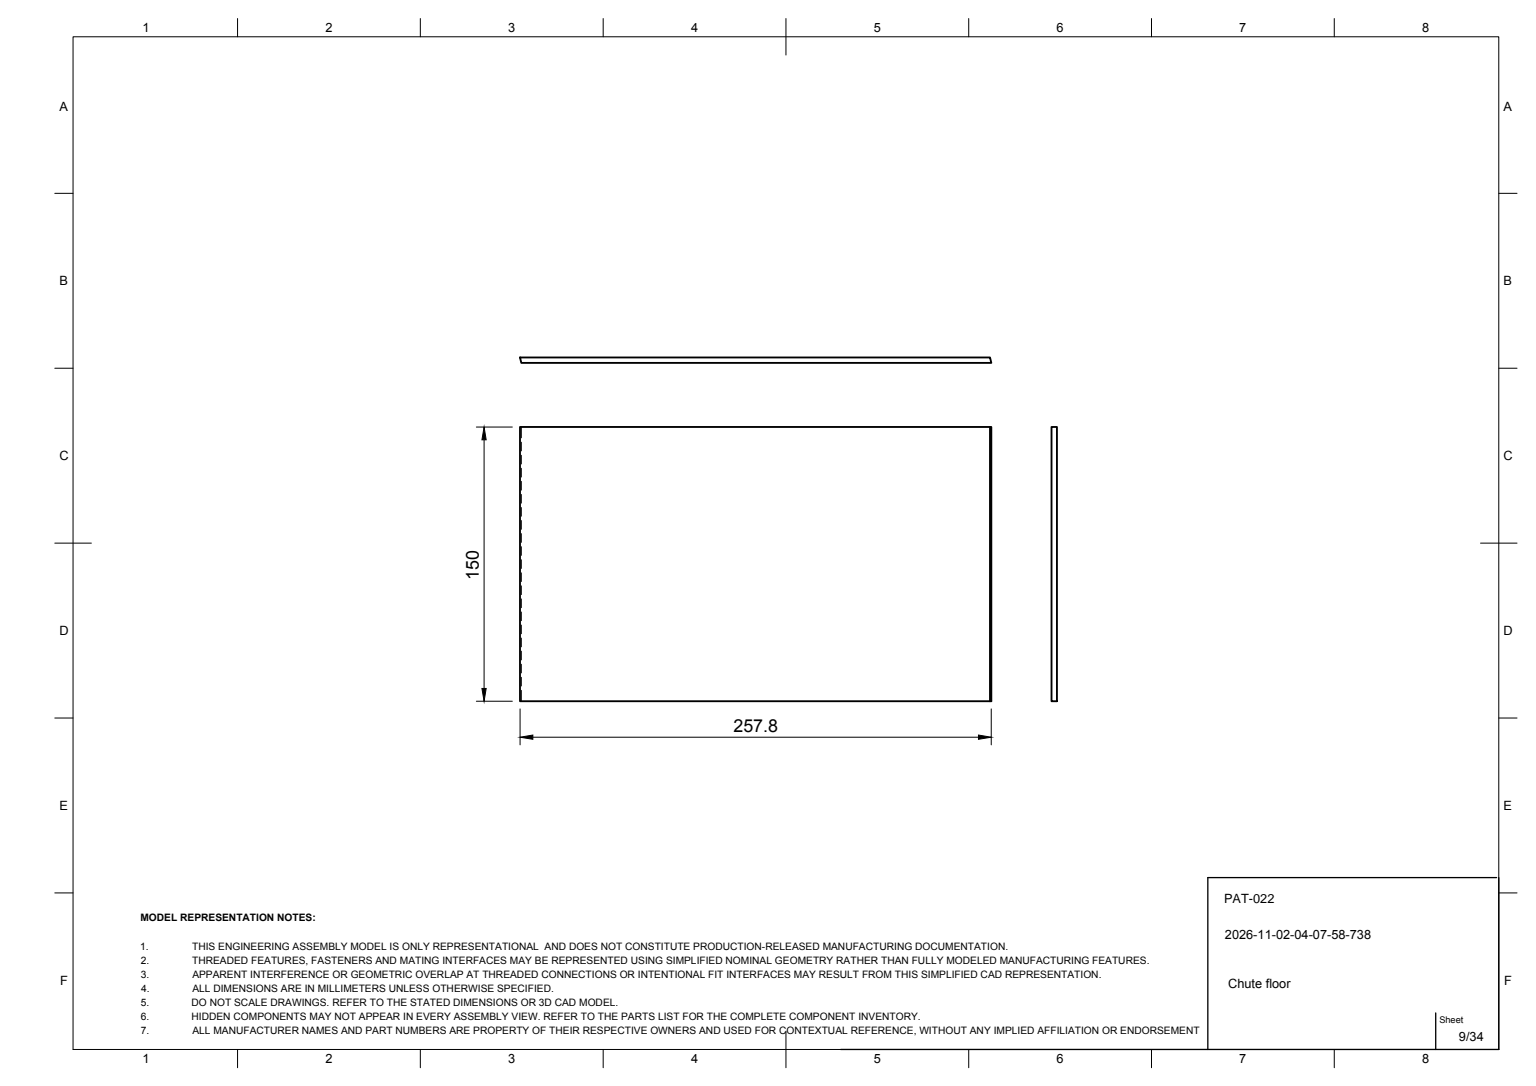
ISO-10303-21;
HEADER;
/* Generated by software containing ST-Developer
 * from STEP Tools, Inc. (www.steptools.com) 
 */

FILE_DESCRIPTION(
/* description */ ('Chute with adjustable gate'),
/* implementation_level */ '2;1');

FILE_NAME(
/* name */ 'Chute floor.step',
/* time_stamp */ '2026-10-27T10:52:28-07:00',
/* author */ (''),
/* organization */ (''),
/* preprocessor_version */ 'ST-DEVELOPER v20.2',
/* originating_system */ 'Autodesk Translation Framework v15.17.0.0',
/* authorisation */ '');

FILE_SCHEMA (('AUTOMOTIVE_DESIGN { 1 0 10303 214 3 1 1 }'));
ENDSEC;

DATA;
#10=MECHANICAL_DESIGN_GEOMETRIC_PRESENTATION_REPRESENTATION('',(#418),#13094);
#354=SHAPE_REPRESENTATION_RELATIONSHIP('SRR','None',#13255,#386);
#386=ADVANCED_BREP_SHAPE_REPRESENTATION('',(#450),#13064);
#418=STYLED_ITEM('',(#13481),#450);
#450=MANIFOLD_SOLID_BREP('Body1',#7601);
#618=PLANE('',#8045);
#619=PLANE('',#8046);
#620=PLANE('',#8047);
#621=PLANE('',#8048);
#622=PLANE('',#8049);
#623=PLANE('',#8050);
#950=FACE_OUTER_BOUND('',#1383,.T.);
#951=FACE_OUTER_BOUND('',#1384,.T.);
#952=FACE_OUTER_BOUND('',#1385,.T.);
#953=FACE_OUTER_BOUND('',#1386,.T.);
#954=FACE_OUTER_BOUND('',#1387,.T.);
#955=FACE_OUTER_BOUND('',#1388,.T.);
#1383=EDGE_LOOP('',(#5354,#5355,#5356,#5357));
#1384=EDGE_LOOP('',(#5358,#5359,#5360,#5361));
#1385=EDGE_LOOP('',(#5362,#5363,#5364,#5365));
#1386=EDGE_LOOP('',(#5366,#5367,#5368,#5369));
#1387=EDGE_LOOP('',(#5370,#5371,#5372,#5373));
#1388=EDGE_LOOP('',(#5374,#5375,#5376,#5377));
#1928=LINE('',#11085,#2705);
#1929=LINE('',#11087,#2706);
#1930=LINE('',#11089,#2707);
#1931=LINE('',#11090,#2708);
#1932=LINE('',#11093,#2709);
#1933=LINE('',#11095,#2710);
#1934=LINE('',#11096,#2711);
#1935=LINE('',#11099,#2712);
#1936=LINE('',#11101,#2713);
#1937=LINE('',#11102,#2714);
#1938=LINE('',#11104,#2715);
#1939=LINE('',#11105,#2716);
#2705=VECTOR('',#8886,1.);
#2706=VECTOR('',#8887,1.);
#2707=VECTOR('',#8888,1.);
#2708=VECTOR('',#8889,1.);
#2709=VECTOR('',#8892,1.);
#2710=VECTOR('',#8893,1.);
#2711=VECTOR('',#8894,1.);
#2712=VECTOR('',#8897,1.);
#2713=VECTOR('',#8898,1.);
#2714=VECTOR('',#8899,1.);
#2715=VECTOR('',#8902,1.);
#2716=VECTOR('',#8903,1.);
#3649=VERTEX_POINT('',#11083);
#3650=VERTEX_POINT('',#11084);
#3651=VERTEX_POINT('',#11086);
#3652=VERTEX_POINT('',#11088);
#3653=VERTEX_POINT('',#11092);
#3654=VERTEX_POINT('',#11094);
#3655=VERTEX_POINT('',#11098);
#3656=VERTEX_POINT('',#11100);
#4310=EDGE_CURVE('',#3649,#3650,#1928,.T.);
#4311=EDGE_CURVE('',#3649,#3651,#1929,.T.);
#4312=EDGE_CURVE('',#3652,#3651,#1930,.T.);
#4313=EDGE_CURVE('',#3650,#3652,#1931,.T.);
#4314=EDGE_CURVE('',#3650,#3653,#1932,.T.);
#4315=EDGE_CURVE('',#3654,#3652,#1933,.T.);
#4316=EDGE_CURVE('',#3653,#3654,#1934,.T.);
#4317=EDGE_CURVE('',#3653,#3655,#1935,.T.);
#4318=EDGE_CURVE('',#3656,#3654,#1936,.T.);
#4319=EDGE_CURVE('',#3655,#3656,#1937,.T.);
#4320=EDGE_CURVE('',#3655,#3649,#1938,.T.);
#4321=EDGE_CURVE('',#3651,#3656,#1939,.T.);
#5354=ORIENTED_EDGE('',*,*,#4310,.F.);
#5355=ORIENTED_EDGE('',*,*,#4311,.T.);
#5356=ORIENTED_EDGE('',*,*,#4312,.F.);
#5357=ORIENTED_EDGE('',*,*,#4313,.F.);
#5358=ORIENTED_EDGE('',*,*,#4314,.F.);
#5359=ORIENTED_EDGE('',*,*,#4313,.T.);
#5360=ORIENTED_EDGE('',*,*,#4315,.F.);
#5361=ORIENTED_EDGE('',*,*,#4316,.F.);
#5362=ORIENTED_EDGE('',*,*,#4317,.F.);
#5363=ORIENTED_EDGE('',*,*,#4316,.T.);
#5364=ORIENTED_EDGE('',*,*,#4318,.F.);
#5365=ORIENTED_EDGE('',*,*,#4319,.F.);
#5366=ORIENTED_EDGE('',*,*,#4320,.F.);
#5367=ORIENTED_EDGE('',*,*,#4319,.T.);
#5368=ORIENTED_EDGE('',*,*,#4321,.F.);
#5369=ORIENTED_EDGE('',*,*,#4311,.F.);
#5370=ORIENTED_EDGE('',*,*,#4321,.T.);
#5371=ORIENTED_EDGE('',*,*,#4318,.T.);
#5372=ORIENTED_EDGE('',*,*,#4315,.T.);
#5373=ORIENTED_EDGE('',*,*,#4312,.T.);
#5374=ORIENTED_EDGE('',*,*,#4320,.T.);
#5375=ORIENTED_EDGE('',*,*,#4310,.T.);
#5376=ORIENTED_EDGE('',*,*,#4314,.T.);
#5377=ORIENTED_EDGE('',*,*,#4317,.T.);
#7218=ADVANCED_FACE('',(#950),#618,.T.);
#7219=ADVANCED_FACE('',(#951),#619,.T.);
#7220=ADVANCED_FACE('',(#952),#620,.T.);
#7221=ADVANCED_FACE('',(#953),#621,.T.);
#7222=ADVANCED_FACE('',(#954),#622,.T.);
#7223=ADVANCED_FACE('',(#955),#623,.F.);
#7601=CLOSED_SHELL('',(#7218,#7219,#7220,#7221,#7222,#7223));
#8044=AXIS2_PLACEMENT_3D('',#11081,#8882,#8883);
#8045=AXIS2_PLACEMENT_3D('',#11082,#8884,#8885);
#8046=AXIS2_PLACEMENT_3D('',#11091,#8890,#8891);
#8047=AXIS2_PLACEMENT_3D('',#11097,#8895,#8896);
#8048=AXIS2_PLACEMENT_3D('',#11103,#8900,#8901);
#8049=AXIS2_PLACEMENT_3D('',#11106,#8904,#8905);
#8050=AXIS2_PLACEMENT_3D('',#11107,#8906,#8907);
#8882=DIRECTION('axis',(0.,0.,1.));
#8883=DIRECTION('refdir',(1.,0.,0.));
#8884=DIRECTION('center_axis',(-1.,0.,0.));
#8885=DIRECTION('ref_axis',(0.,0.,1.));
#8886=DIRECTION('',(0.,0.,-1.));
#8887=DIRECTION('',(0.,1.,0.));
#8888=DIRECTION('',(0.,0.,1.));
#8889=DIRECTION('',(0.,1.,0.));
#8890=DIRECTION('center_axis',(0.233372952475324,0.,-0.972387301980517));
#8891=DIRECTION('ref_axis',(-0.972387301980517,0.,-0.233372952475324));
#8892=DIRECTION('',(0.972387301980517,0.,0.233372952475324));
#8893=DIRECTION('',(-0.972387301980517,0.,-0.233372952475324));
#8894=DIRECTION('',(0.,1.,0.));
#8895=DIRECTION('center_axis',(1.,0.,0.));
#8896=DIRECTION('ref_axis',(0.,0.,-1.));
#8897=DIRECTION('',(0.,0.,1.));
#8898=DIRECTION('',(0.,0.,-1.));
#8899=DIRECTION('',(0.,1.,0.));
#8900=DIRECTION('center_axis',(-0.233372952475324,0.,0.972387301980517));
#8901=DIRECTION('ref_axis',(0.972387301980517,0.,0.233372952475324));
#8902=DIRECTION('',(-0.972387301980517,0.,-0.233372952475324));
#8903=DIRECTION('',(0.972387301980517,0.,0.233372952475324));
#8904=DIRECTION('center_axis',(0.,1.,0.));
#8905=DIRECTION('ref_axis',(0.,0.,1.));
#8906=DIRECTION('center_axis',(0.,1.,0.));
#8907=DIRECTION('ref_axis',(1.,0.,0.));
#11081=CARTESIAN_POINT('',(0.,0.,0.));
#11082=CARTESIAN_POINT('Origin',(0.,-7.5,4.));
#11083=CARTESIAN_POINT('',(0.,-7.5,4.3));
#11084=CARTESIAN_POINT('',(0.,-7.5,4.));
#11085=CARTESIAN_POINT('',(0.,-7.5,4.3));
#11086=CARTESIAN_POINT('',(0.,7.5,4.3));
#11087=CARTESIAN_POINT('',(0.,-7.5,4.3));
#11088=CARTESIAN_POINT('',(0.,7.5,4.));
#11089=CARTESIAN_POINT('',(0.,7.5,4.3));
#11090=CARTESIAN_POINT('',(0.,-7.5,4.));
#11091=CARTESIAN_POINT('Origin',(25.,-7.5,10.));
#11092=CARTESIAN_POINT('',(25.,-7.5,10.));
#11093=CARTESIAN_POINT('',(0.,-7.5,4.));
#11094=CARTESIAN_POINT('',(25.,7.5,10.));
#11095=CARTESIAN_POINT('',(0.,7.5,4.));
#11096=CARTESIAN_POINT('',(25.,-7.5,10.));
#11097=CARTESIAN_POINT('Origin',(25.,-7.5,10.3));
#11098=CARTESIAN_POINT('',(25.,-7.5,10.3));
#11099=CARTESIAN_POINT('',(25.,-7.5,10.));
#11100=CARTESIAN_POINT('',(25.,7.5,10.3));
#11101=CARTESIAN_POINT('',(25.,7.5,10.));
#11102=CARTESIAN_POINT('',(25.,-7.5,10.3));
#11103=CARTESIAN_POINT('Origin',(0.,-7.5,4.3));
#11104=CARTESIAN_POINT('',(25.,-7.5,10.3));
#11105=CARTESIAN_POINT('',(25.,7.5,10.3));
#11106=CARTESIAN_POINT('Origin',(12.5,7.5,7.15));
#11107=CARTESIAN_POINT('Origin',(12.5,-7.5,7.15));
#13027=UNCERTAINTY_MEASURE_WITH_UNIT(LENGTH_MEASURE(0.001),#13095,
'DISTANCE_ACCURACY_VALUE',
'Maximum model space distance between geometric entities at asserted c
onnectivities');
#13057=UNCERTAINTY_MEASURE_WITH_UNIT(LENGTH_MEASURE(0.001),#13095,
'DISTANCE_ACCURACY_VALUE',
'Maximum model space distance between geometric entities at asserted c
onnectivities');
#13064=(
GEOMETRIC_REPRESENTATION_CONTEXT(3)
GLOBAL_UNCERTAINTY_ASSIGNED_CONTEXT((#13027))
GLOBAL_UNIT_ASSIGNED_CONTEXT((#13095,#13097,#13098))
REPRESENTATION_CONTEXT('','3D')
);
#13094=(
GEOMETRIC_REPRESENTATION_CONTEXT(3)
GLOBAL_UNCERTAINTY_ASSIGNED_CONTEXT((#13057))
GLOBAL_UNIT_ASSIGNED_CONTEXT((#13095,#13097,#13098))
REPRESENTATION_CONTEXT('','3D')
);
#13095=(
LENGTH_UNIT()
NAMED_UNIT(*)
SI_UNIT(.CENTI.,.METRE.)
);
#13097=(
NAMED_UNIT(*)
PLANE_ANGLE_UNIT()
SI_UNIT($,.RADIAN.)
);
#13098=(
NAMED_UNIT(*)
SI_UNIT($,.STERADIAN.)
SOLID_ANGLE_UNIT()
);
#13105=SHAPE_DEFINITION_REPRESENTATION(#13141,#13255);
#13141=PRODUCT_DEFINITION_SHAPE('',$,#13292);
#13255=SHAPE_REPRESENTATION('',(#8044),#13064);
#13285=PRODUCT_DEFINITION_CONTEXT('part definition',#13395,'design');
#13292=PRODUCT_DEFINITION('Chute floor','Chute floor',#13328,#13285);
#13328=PRODUCT_DEFINITION_FORMATION('',$,#13403);
#13395=APPLICATION_CONTEXT(
'Core Data for Automotive Mechanical Design Process');
#13396=PRODUCT_CONTEXT('part definition',#13395,'mechanical');
#13403=PRODUCT('Chute floor','Chute floor','Chute floor',(#13396));
#13475=COLOUR_RGB('Light Blue',0.38,0.62,0.78);
#13476=FILL_AREA_STYLE_COLOUR('',#13475);
#13477=FILL_AREA_STYLE('',(#13476));
#13478=SURFACE_STYLE_FILL_AREA(#13477);
#13479=SURFACE_SIDE_STYLE('',(#13478));
#13480=SURFACE_STYLE_USAGE(.BOTH.,#13479);
#13481=PRESENTATION_STYLE_ASSIGNMENT((#13480));
ENDSEC;
END-ISO-10303-21;
